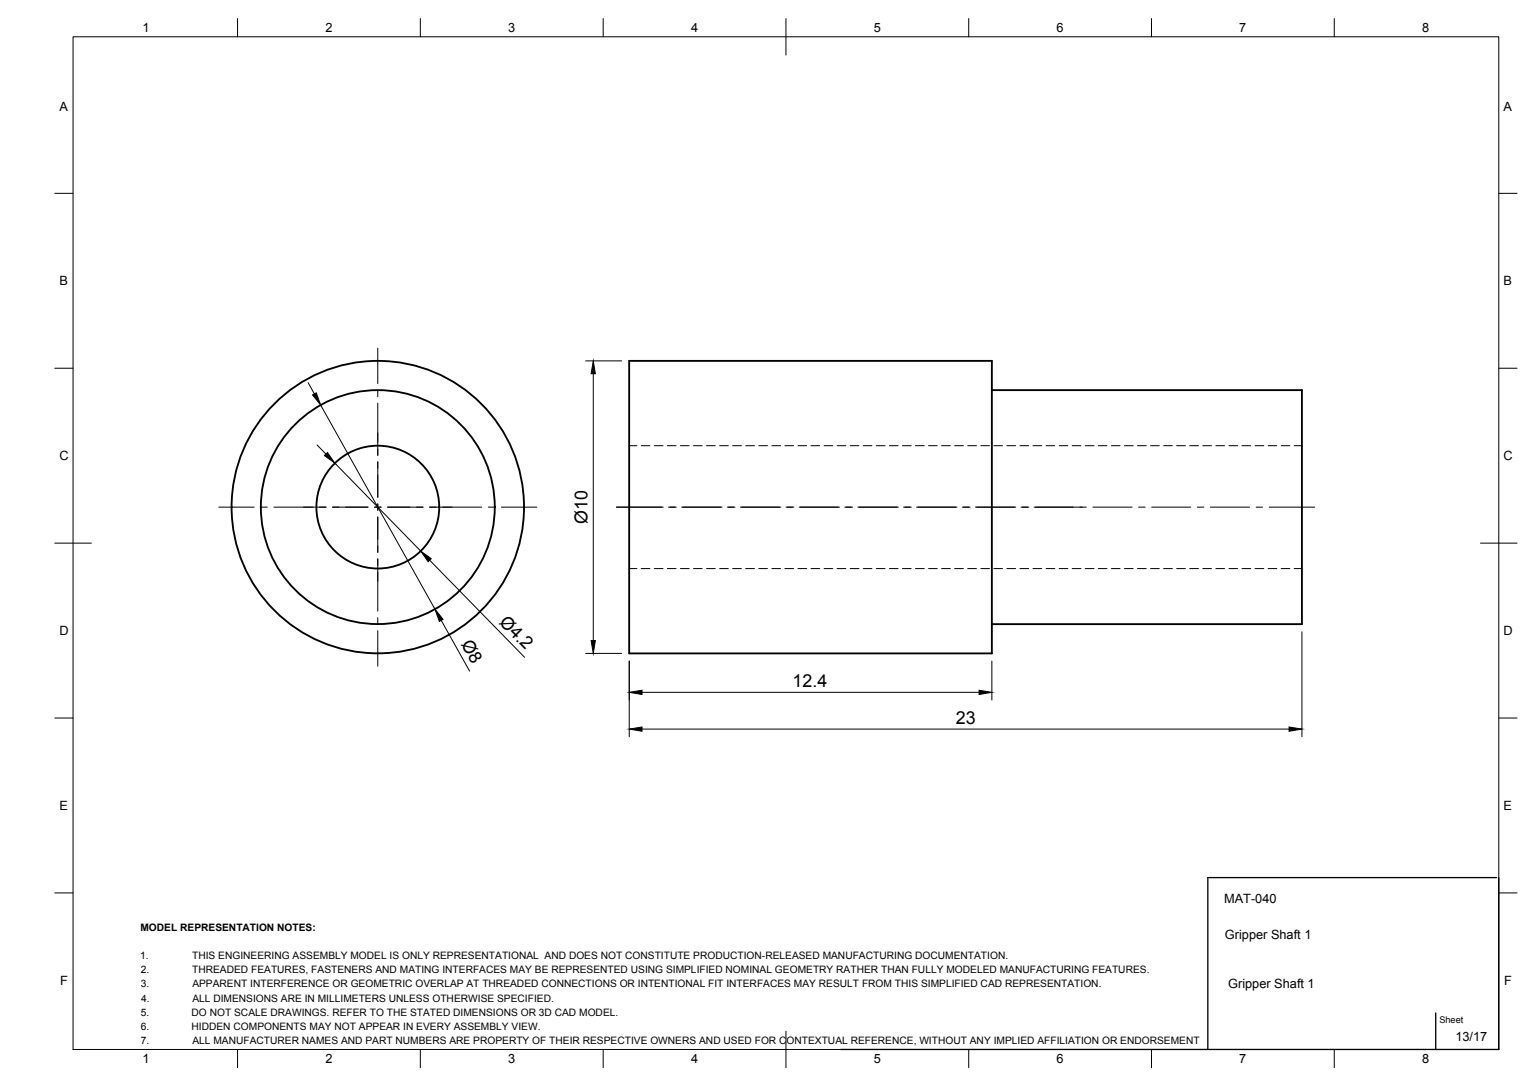
ISO-10303-21;
HEADER;
/* Generated by software containing ST-Developer
 * from STEP Tools, Inc. (www.steptools.com) 
 */

FILE_DESCRIPTION(
/* description */ ('STEP AP214'),
/* implementation_level */ '2;1');

FILE_NAME(
/* name */ 'Gripper Shaft 1.step',
/* time_stamp */ '2026-11-14T21:53:28-08:00',
/* author */ (''),
/* organization */ (''),
/* preprocessor_version */ 'ST-DEVELOPER v20.2',
/* originating_system */ 'Autodesk Translation Framework v15.17.0.0',
/* authorisation */ '');

FILE_SCHEMA (('AUTOMOTIVE_DESIGN { 1 0 10303 214 3 1 1 }'));
ENDSEC;

DATA;
#10=MECHANICAL_DESIGN_GEOMETRIC_PRESENTATION_REPRESENTATION('',(#349),#20176);
#302=SHAPE_REPRESENTATION_RELATIONSHIP('SRR','None',#20266,#314);
#314=ADVANCED_BREP_SHAPE_REPRESENTATION('',(#376),#20172);
#349=STYLED_ITEM('',(#20337),#376);
#376=MANIFOLD_SOLID_BREP('Body1',#10967);
#565=FACE_BOUND('',#2231,.T.);
#566=FACE_BOUND('',#2233,.T.);
#567=FACE_BOUND('',#2235,.T.);
#876=PLANE('',#12099);
#877=PLANE('',#12100);
#878=PLANE('',#12101);
#1450=FACE_OUTER_BOUND('',#2227,.T.);
#1451=FACE_OUTER_BOUND('',#2228,.T.);
#1452=FACE_OUTER_BOUND('',#2229,.T.);
#1453=FACE_OUTER_BOUND('',#2230,.T.);
#1454=FACE_OUTER_BOUND('',#2232,.T.);
#1455=FACE_OUTER_BOUND('',#2234,.T.);
#2227=EDGE_LOOP('',(#9981,#9982,#9983,#9984));
#2228=EDGE_LOOP('',(#9985,#9986,#9987,#9988));
#2229=EDGE_LOOP('',(#9989,#9990,#9991,#9992));
#2230=EDGE_LOOP('',(#9993));
#2231=EDGE_LOOP('',(#9994));
#2232=EDGE_LOOP('',(#9995));
#2233=EDGE_LOOP('',(#9996));
#2234=EDGE_LOOP('',(#9997));
#2235=EDGE_LOOP('',(#9998));
#3221=LINE('',#19927,#4209);
#3222=LINE('',#19933,#4210);
#3223=LINE('',#19939,#4211);
#4209=VECTOR('',#15131,5.);
#4210=VECTOR('',#15138,2.1);
#4211=VECTOR('',#15145,4.);
#4692=CIRCLE('',#12091,5.);
#4693=CIRCLE('',#12092,5.);
#4694=CIRCLE('',#12094,2.1);
#4695=CIRCLE('',#12095,2.1);
#4696=CIRCLE('',#12097,4.);
#4697=CIRCLE('',#12098,4.);
#5643=VERTEX_POINT('',#19924);
#5644=VERTEX_POINT('',#19926);
#5645=VERTEX_POINT('',#19930);
#5646=VERTEX_POINT('',#19932);
#5647=VERTEX_POINT('',#19936);
#5648=VERTEX_POINT('',#19938);
#7101=EDGE_CURVE('',#5643,#5643,#4692,.T.);
#7102=EDGE_CURVE('',#5643,#5644,#3221,.T.);
#7103=EDGE_CURVE('',#5644,#5644,#4693,.T.);
#7104=EDGE_CURVE('',#5645,#5645,#4694,.T.);
#7105=EDGE_CURVE('',#5645,#5646,#3222,.T.);
#7106=EDGE_CURVE('',#5646,#5646,#4695,.T.);
#7107=EDGE_CURVE('',#5647,#5647,#4696,.T.);
#7108=EDGE_CURVE('',#5647,#5648,#3223,.T.);
#7109=EDGE_CURVE('',#5648,#5648,#4697,.T.);
#9981=ORIENTED_EDGE('',*,*,#7101,.F.);
#9982=ORIENTED_EDGE('',*,*,#7102,.T.);
#9983=ORIENTED_EDGE('',*,*,#7103,.T.);
#9984=ORIENTED_EDGE('',*,*,#7102,.F.);
#9985=ORIENTED_EDGE('',*,*,#7104,.T.);
#9986=ORIENTED_EDGE('',*,*,#7105,.T.);
#9987=ORIENTED_EDGE('',*,*,#7106,.F.);
#9988=ORIENTED_EDGE('',*,*,#7105,.F.);
#9989=ORIENTED_EDGE('',*,*,#7107,.F.);
#9990=ORIENTED_EDGE('',*,*,#7108,.T.);
#9991=ORIENTED_EDGE('',*,*,#7109,.F.);
#9992=ORIENTED_EDGE('',*,*,#7108,.F.);
#9993=ORIENTED_EDGE('',*,*,#7109,.T.);
#9994=ORIENTED_EDGE('',*,*,#7104,.F.);
#9995=ORIENTED_EDGE('',*,*,#7101,.T.);
#9996=ORIENTED_EDGE('',*,*,#7106,.T.);
#9997=ORIENTED_EDGE('',*,*,#7103,.F.);
#9998=ORIENTED_EDGE('',*,*,#7107,.T.);
#10340=CYLINDRICAL_SURFACE('',#12090,5.);
#10341=CYLINDRICAL_SURFACE('',#12093,2.1);
#10342=CYLINDRICAL_SURFACE('',#12096,4.);
#10902=ADVANCED_FACE('',(#1450),#10340,.T.);
#10903=ADVANCED_FACE('',(#1451),#10341,.F.);
#10904=ADVANCED_FACE('',(#1452),#10342,.T.);
#10905=ADVANCED_FACE('',(#1453,#565),#876,.T.);
#10906=ADVANCED_FACE('',(#1454,#566),#877,.F.);
#10907=ADVANCED_FACE('',(#1455,#567),#878,.F.);
#10967=CLOSED_SHELL('',(#10902,#10903,#10904,#10905,#10906,#10907));
#12089=AXIS2_PLACEMENT_3D('',#19922,#15125,#15126);
#12090=AXIS2_PLACEMENT_3D('',#19923,#15127,#15128);
#12091=AXIS2_PLACEMENT_3D('',#19925,#15129,#15130);
#12092=AXIS2_PLACEMENT_3D('',#19928,#15132,#15133);
#12093=AXIS2_PLACEMENT_3D('',#19929,#15134,#15135);
#12094=AXIS2_PLACEMENT_3D('',#19931,#15136,#15137);
#12095=AXIS2_PLACEMENT_3D('',#19934,#15139,#15140);
#12096=AXIS2_PLACEMENT_3D('',#19935,#15141,#15142);
#12097=AXIS2_PLACEMENT_3D('',#19937,#15143,#15144);
#12098=AXIS2_PLACEMENT_3D('',#19940,#15146,#15147);
#12099=AXIS2_PLACEMENT_3D('',#19941,#15148,#15149);
#12100=AXIS2_PLACEMENT_3D('',#19942,#15150,#15151);
#12101=AXIS2_PLACEMENT_3D('',#19943,#15152,#15153);
#15125=DIRECTION('axis',(0.,0.,1.));
#15126=DIRECTION('refdir',(1.,0.,0.));
#15127=DIRECTION('center_axis',(0.,0.,-1.));
#15128=DIRECTION('ref_axis',(-1.,0.,0.));
#15129=DIRECTION('center_axis',(0.,0.,-1.));
#15130=DIRECTION('ref_axis',(-1.,0.,0.));
#15131=DIRECTION('',(0.,0.,1.));
#15132=DIRECTION('center_axis',(0.,0.,-1.));
#15133=DIRECTION('ref_axis',(-1.,0.,0.));
#15134=DIRECTION('center_axis',(0.,0.,-1.));
#15135=DIRECTION('ref_axis',(-1.,0.,0.));
#15136=DIRECTION('center_axis',(0.,0.,1.));
#15137=DIRECTION('ref_axis',(1.,0.,0.));
#15138=DIRECTION('',(0.,0.,-1.));
#15139=DIRECTION('center_axis',(0.,0.,1.));
#15140=DIRECTION('ref_axis',(1.,0.,0.));
#15141=DIRECTION('center_axis',(0.,0.,-1.));
#15142=DIRECTION('ref_axis',(-1.,0.,0.));
#15143=DIRECTION('center_axis',(0.,0.,-1.));
#15144=DIRECTION('ref_axis',(-1.,0.,0.));
#15145=DIRECTION('',(0.,0.,1.));
#15146=DIRECTION('center_axis',(0.,0.,1.));
#15147=DIRECTION('ref_axis',(1.,0.,0.));
#15148=DIRECTION('center_axis',(0.,0.,1.));
#15149=DIRECTION('ref_axis',(1.,0.,0.));
#15150=DIRECTION('center_axis',(0.,0.,1.));
#15151=DIRECTION('ref_axis',(1.,0.,0.));
#15152=DIRECTION('center_axis',(0.,0.,-1.));
#15153=DIRECTION('ref_axis',(-1.,0.,0.));
#19922=CARTESIAN_POINT('',(0.,0.,0.));
#19923=CARTESIAN_POINT('Origin',(0.,0.,12.4));
#19924=CARTESIAN_POINT('',(5.,-6.12323399573677E-16,0.));
#19925=CARTESIAN_POINT('Origin',(0.,0.,0.));
#19926=CARTESIAN_POINT('',(5.,-6.12323399573677E-16,12.4));
#19927=CARTESIAN_POINT('',(5.,-6.12323399573677E-16,12.4));
#19928=CARTESIAN_POINT('Origin',(0.,0.,12.4));
#19929=CARTESIAN_POINT('Origin',(0.,0.,23.));
#19930=CARTESIAN_POINT('',(2.1,-2.57175827820944E-16,23.));
#19931=CARTESIAN_POINT('Origin',(0.,0.,23.));
#19932=CARTESIAN_POINT('',(2.1,-2.57175827820944E-16,0.));
#19933=CARTESIAN_POINT('',(2.1,-2.57175827820944E-16,23.));
#19934=CARTESIAN_POINT('Origin',(0.,0.,0.));
#19935=CARTESIAN_POINT('Origin',(0.,0.,23.));
#19936=CARTESIAN_POINT('',(4.,-4.89858719658941E-16,12.4));
#19937=CARTESIAN_POINT('Origin',(0.,0.,12.4));
#19938=CARTESIAN_POINT('',(4.,-4.89858719658941E-16,23.));
#19939=CARTESIAN_POINT('',(4.,-4.89858719658941E-16,23.));
#19940=CARTESIAN_POINT('Origin',(0.,0.,23.));
#19941=CARTESIAN_POINT('Origin',(0.,0.,23.));
#19942=CARTESIAN_POINT('Origin',(0.,0.,0.));
#19943=CARTESIAN_POINT('Origin',(0.,0.,12.4));
#20156=UNCERTAINTY_MEASURE_WITH_UNIT(LENGTH_MEASURE(0.01),#20177,
'DISTANCE_ACCURACY_VALUE',
'Maximum model space distance between geometric entities at asserted c
onnectivities');
#20160=UNCERTAINTY_MEASURE_WITH_UNIT(LENGTH_MEASURE(0.01),#20177,
'DISTANCE_ACCURACY_VALUE',
'Maximum model space distance between geometric entities at asserted c
onnectivities');
#20172=(
GEOMETRIC_REPRESENTATION_CONTEXT(3)
GLOBAL_UNCERTAINTY_ASSIGNED_CONTEXT((#20156))
GLOBAL_UNIT_ASSIGNED_CONTEXT((#20177,#20179,#20180))
REPRESENTATION_CONTEXT('','3D')
);
#20176=(
GEOMETRIC_REPRESENTATION_CONTEXT(3)
GLOBAL_UNCERTAINTY_ASSIGNED_CONTEXT((#20160))
GLOBAL_UNIT_ASSIGNED_CONTEXT((#20177,#20179,#20180))
REPRESENTATION_CONTEXT('','3D')
);
#20177=(
LENGTH_UNIT()
NAMED_UNIT(*)
SI_UNIT(.MILLI.,.METRE.)
);
#20179=(
NAMED_UNIT(*)
PLANE_ANGLE_UNIT()
SI_UNIT($,.RADIAN.)
);
#20180=(
NAMED_UNIT(*)
SI_UNIT($,.STERADIAN.)
SOLID_ANGLE_UNIT()
);
#20192=SHAPE_DEFINITION_REPRESENTATION(#20207,#20266);
#20207=PRODUCT_DEFINITION_SHAPE('',$,#20282);
#20266=SHAPE_REPRESENTATION('',(#12089),#20172);
#20270=PRODUCT_DEFINITION_CONTEXT('part definition',#20317,'design');
#20282=PRODUCT_DEFINITION('Gripper Shaft 1','Gripper Shaft 1',#20297,#20270);
#20297=PRODUCT_DEFINITION_FORMATION('',$,#20330);
#20317=APPLICATION_CONTEXT(
'Core Data for Automotive Mechanical Design Process');
#20318=PRODUCT_CONTEXT('part definition',#20317,'mechanical');
#20330=PRODUCT('Gripper Shaft 1','Gripper Shaft 1',$,(#20318));
#20337=PRESENTATION_STYLE_ASSIGNMENT((#20342));
#20342=SURFACE_STYLE_USAGE(.BOTH.,#20347);
#20347=SURFACE_SIDE_STYLE('',(#20352));
#20352=SURFACE_STYLE_FILL_AREA(#20357);
#20357=FILL_AREA_STYLE('Opaque(31,36,43)',(#20362));
#20362=FILL_AREA_STYLE_COLOUR('Opaque(31,36,43)',#20367);
#20367=COLOUR_RGB('Opaque(31,36,43)',0.12156862745098,0.141176470588235,
0.168627450980392);
ENDSEC;
END-ISO-10303-21;
